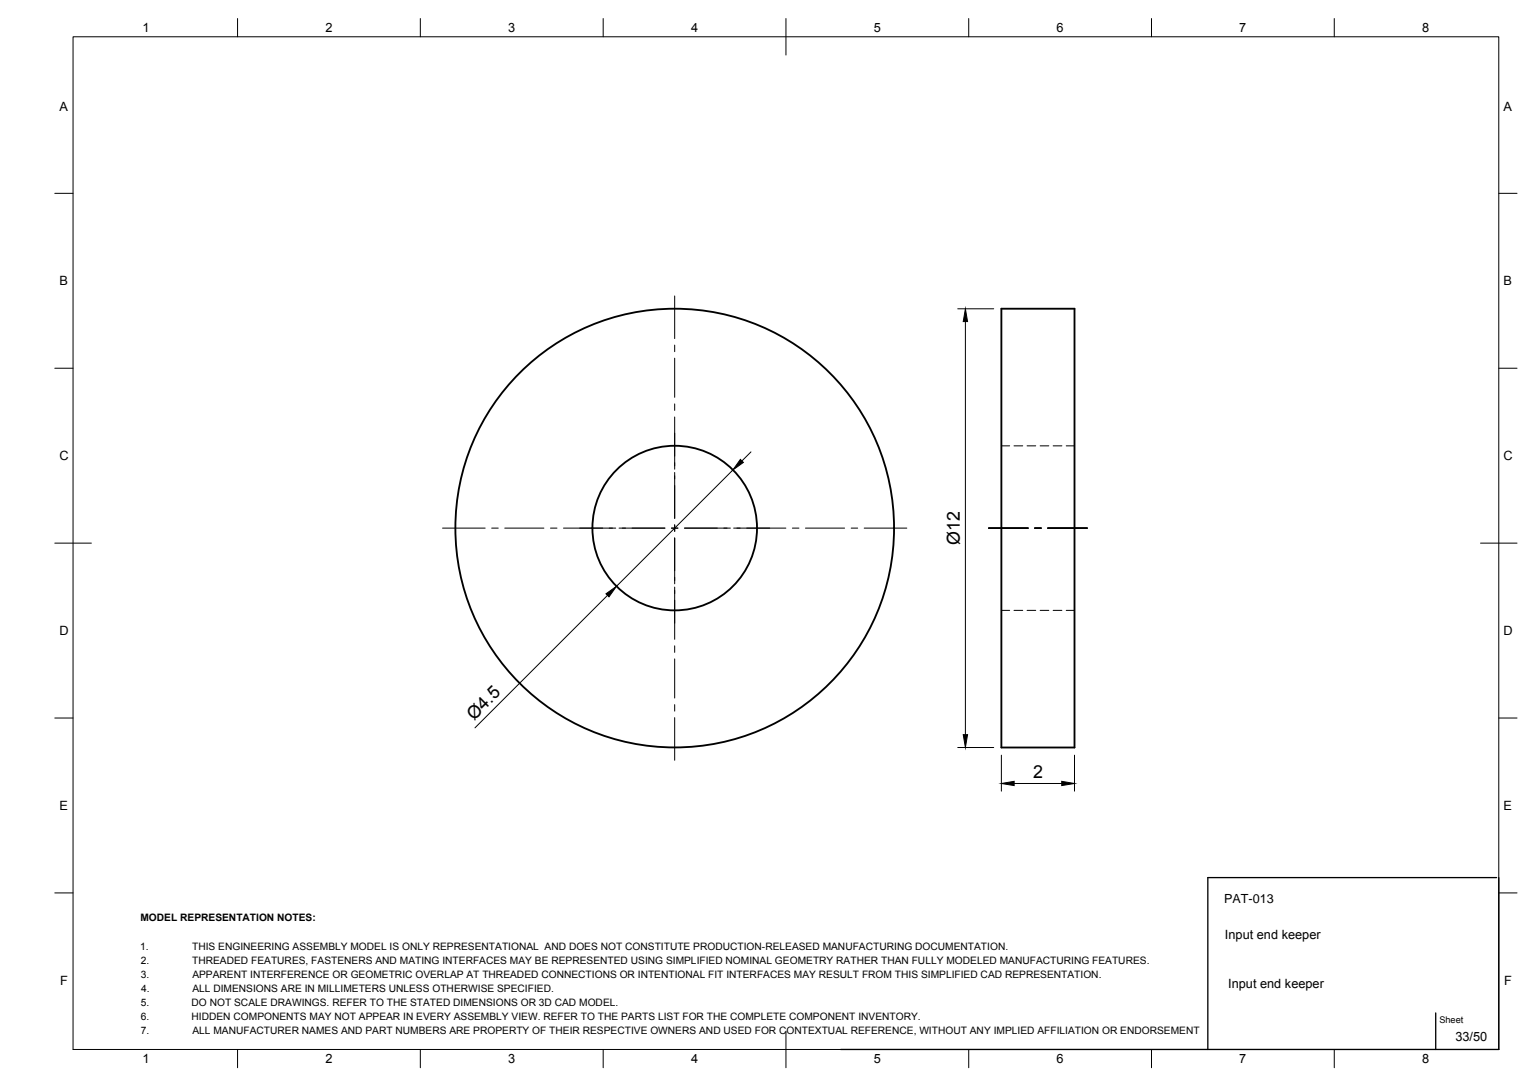
ISO-10303-21;
HEADER;
/* Generated by software containing ST-Developer
 * from STEP Tools, Inc. (www.steptools.com) 
 */

FILE_DESCRIPTION(
/* description */ ('Belt-driven linear axis on 2020 extrusion'),
/* implementation_level */ '2;1');

FILE_NAME(
/* name */ 'Input end keeper.step',
/* time_stamp */ '2026-10-28T03:26:09-07:00',
/* author */ (''),
/* organization */ (''),
/* preprocessor_version */ 'ST-DEVELOPER v20.2',
/* originating_system */ 'Autodesk Translation Framework v15.17.0.0',
/* authorisation */ '');

FILE_SCHEMA (('AUTOMOTIVE_DESIGN { 1 0 10303 214 3 1 1 }'));
ENDSEC;

DATA;
#10=MECHANICAL_DESIGN_GEOMETRIC_PRESENTATION_REPRESENTATION('',(#648),#20096);
#546=SHAPE_REPRESENTATION_RELATIONSHIP('SRR','None',#20344,#592);
#592=ADVANCED_BREP_SHAPE_REPRESENTATION('',(#703),#20075);
#648=STYLED_ITEM('',(#20643),#703);
#703=MANIFOLD_SOLID_BREP('Body1',#10962);
#838=FACE_BOUND('',#2390,.T.);
#839=FACE_BOUND('',#2392,.T.);
#1125=PLANE('',#12252);
#1126=PLANE('',#12253);
#1645=FACE_OUTER_BOUND('',#2387,.T.);
#1646=FACE_OUTER_BOUND('',#2388,.T.);
#1647=FACE_OUTER_BOUND('',#2389,.T.);
#1648=FACE_OUTER_BOUND('',#2391,.T.);
#2387=EDGE_LOOP('',(#9037,#9038,#9039,#9040));
#2388=EDGE_LOOP('',(#9041,#9042,#9043,#9044));
#2389=EDGE_LOOP('',(#9045));
#2390=EDGE_LOOP('',(#9046));
#2391=EDGE_LOOP('',(#9047));
#2392=EDGE_LOOP('',(#9048));
#3216=LINE('',#18502,#4073);
#3217=LINE('',#18508,#4074);
#4073=VECTOR('',#14852,0.225);
#4074=VECTOR('',#14859,0.6);
#4700=CIRCLE('',#12247,0.225);
#4701=CIRCLE('',#12248,0.225);
#4702=CIRCLE('',#12250,0.6);
#4703=CIRCLE('',#12251,0.6);
#5495=VERTEX_POINT('',#18499);
#5496=VERTEX_POINT('',#18501);
#5497=VERTEX_POINT('',#18505);
#5498=VERTEX_POINT('',#18507);
#6733=EDGE_CURVE('',#5495,#5495,#4700,.T.);
#6734=EDGE_CURVE('',#5495,#5496,#3216,.T.);
#6735=EDGE_CURVE('',#5496,#5496,#4701,.T.);
#6736=EDGE_CURVE('',#5497,#5497,#4702,.T.);
#6737=EDGE_CURVE('',#5497,#5498,#3217,.T.);
#6738=EDGE_CURVE('',#5498,#5498,#4703,.T.);
#9037=ORIENTED_EDGE('',*,*,#6733,.F.);
#9038=ORIENTED_EDGE('',*,*,#6734,.T.);
#9039=ORIENTED_EDGE('',*,*,#6735,.T.);
#9040=ORIENTED_EDGE('',*,*,#6734,.F.);
#9041=ORIENTED_EDGE('',*,*,#6736,.F.);
#9042=ORIENTED_EDGE('',*,*,#6737,.T.);
#9043=ORIENTED_EDGE('',*,*,#6738,.T.);
#9044=ORIENTED_EDGE('',*,*,#6737,.F.);
#9045=ORIENTED_EDGE('',*,*,#6736,.T.);
#9046=ORIENTED_EDGE('',*,*,#6733,.T.);
#9047=ORIENTED_EDGE('',*,*,#6738,.F.);
#9048=ORIENTED_EDGE('',*,*,#6735,.F.);
#10211=CYLINDRICAL_SURFACE('',#12246,0.225);
#10212=CYLINDRICAL_SURFACE('',#12249,0.6);
#10696=ADVANCED_FACE('',(#1645),#10211,.F.);
#10697=ADVANCED_FACE('',(#1646),#10212,.T.);
#10698=ADVANCED_FACE('',(#1647,#838),#1125,.T.);
#10699=ADVANCED_FACE('',(#1648,#839),#1126,.F.);
#10962=CLOSED_SHELL('',(#10696,#10697,#10698,#10699));
#12245=AXIS2_PLACEMENT_3D('',#18497,#14846,#14847);
#12246=AXIS2_PLACEMENT_3D('',#18498,#14848,#14849);
#12247=AXIS2_PLACEMENT_3D('',#18500,#14850,#14851);
#12248=AXIS2_PLACEMENT_3D('',#18503,#14853,#14854);
#12249=AXIS2_PLACEMENT_3D('',#18504,#14855,#14856);
#12250=AXIS2_PLACEMENT_3D('',#18506,#14857,#14858);
#12251=AXIS2_PLACEMENT_3D('',#18509,#14860,#14861);
#12252=AXIS2_PLACEMENT_3D('',#18510,#14862,#14863);
#12253=AXIS2_PLACEMENT_3D('',#18511,#14864,#14865);
#14846=DIRECTION('axis',(0.,0.,1.));
#14847=DIRECTION('refdir',(1.,0.,0.));
#14848=DIRECTION('center_axis',(0.,1.,0.));
#14849=DIRECTION('ref_axis',(1.,0.,0.));
#14850=DIRECTION('center_axis',(0.,-1.,0.));
#14851=DIRECTION('ref_axis',(1.,0.,0.));
#14852=DIRECTION('',(0.,-1.,0.));
#14853=DIRECTION('center_axis',(0.,-1.,0.));
#14854=DIRECTION('ref_axis',(1.,0.,0.));
#14855=DIRECTION('center_axis',(0.,1.,0.));
#14856=DIRECTION('ref_axis',(1.,0.,0.));
#14857=DIRECTION('center_axis',(0.,1.,0.));
#14858=DIRECTION('ref_axis',(1.,0.,0.));
#14859=DIRECTION('',(0.,-1.,0.));
#14860=DIRECTION('center_axis',(0.,1.,0.));
#14861=DIRECTION('ref_axis',(1.,0.,0.));
#14862=DIRECTION('center_axis',(0.,1.,0.));
#14863=DIRECTION('ref_axis',(1.,0.,0.));
#14864=DIRECTION('center_axis',(0.,1.,0.));
#14865=DIRECTION('ref_axis',(1.,0.,0.));
#18497=CARTESIAN_POINT('',(0.,0.,0.));
#18498=CARTESIAN_POINT('Origin',(0.,-5.2,7.));
#18499=CARTESIAN_POINT('',(-0.225,-5.,7.));
#18500=CARTESIAN_POINT('Origin',(0.,-5.,7.));
#18501=CARTESIAN_POINT('',(-0.225,-5.2,7.));
#18502=CARTESIAN_POINT('',(-0.225,-5.2,7.));
#18503=CARTESIAN_POINT('Origin',(0.,-5.2,7.));
#18504=CARTESIAN_POINT('Origin',(0.,-5.2,7.));
#18505=CARTESIAN_POINT('',(-0.6,-5.,7.));
#18506=CARTESIAN_POINT('Origin',(0.,-5.,7.));
#18507=CARTESIAN_POINT('',(-0.6,-5.2,7.));
#18508=CARTESIAN_POINT('',(-0.6,-5.2,7.));
#18509=CARTESIAN_POINT('Origin',(0.,-5.2,7.));
#18510=CARTESIAN_POINT('Origin',(0.,-5.,7.));
#18511=CARTESIAN_POINT('Origin',(0.,-5.2,7.));
#20021=UNCERTAINTY_MEASURE_WITH_UNIT(LENGTH_MEASURE(0.001),#20097,
'DISTANCE_ACCURACY_VALUE',
'Maximum model space distance between geometric entities at asserted c
onnectivities');
#20042=UNCERTAINTY_MEASURE_WITH_UNIT(LENGTH_MEASURE(0.001),#20097,
'DISTANCE_ACCURACY_VALUE',
'Maximum model space distance between geometric entities at asserted c
onnectivities');
#20075=(
GEOMETRIC_REPRESENTATION_CONTEXT(3)
GLOBAL_UNCERTAINTY_ASSIGNED_CONTEXT((#20021))
GLOBAL_UNIT_ASSIGNED_CONTEXT((#20097,#20099,#20100))
REPRESENTATION_CONTEXT('','3D')
);
#20096=(
GEOMETRIC_REPRESENTATION_CONTEXT(3)
GLOBAL_UNCERTAINTY_ASSIGNED_CONTEXT((#20042))
GLOBAL_UNIT_ASSIGNED_CONTEXT((#20097,#20099,#20100))
REPRESENTATION_CONTEXT('','3D')
);
#20097=(
LENGTH_UNIT()
NAMED_UNIT(*)
SI_UNIT(.CENTI.,.METRE.)
);
#20099=(
NAMED_UNIT(*)
PLANE_ANGLE_UNIT()
SI_UNIT($,.RADIAN.)
);
#20100=(
NAMED_UNIT(*)
SI_UNIT($,.STERADIAN.)
SOLID_ANGLE_UNIT()
);
#20133=SHAPE_DEFINITION_REPRESENTATION(#20191,#20344);
#20191=PRODUCT_DEFINITION_SHAPE('',$,#20398);
#20344=SHAPE_REPRESENTATION('',(#12245),#20075);
#20365=PRODUCT_DEFINITION_CONTEXT('part definition',#20526,'design');
#20398=PRODUCT_DEFINITION('Input end keeper','Input end keeper',#20451,
#20365);
#20451=PRODUCT_DEFINITION_FORMATION('',$,#20560);
#20526=APPLICATION_CONTEXT(
'Core Data for Automotive Mechanical Design Process');
#20527=PRODUCT_CONTEXT('part definition',#20526,'mechanical');
#20560=PRODUCT('Input end keeper','Input end keeper','Input end keeper',
(#20527));
#20637=COLOUR_RGB('Sky Blue',0.24,0.69,0.87);
#20638=FILL_AREA_STYLE_COLOUR('',#20637);
#20639=FILL_AREA_STYLE('',(#20638));
#20640=SURFACE_STYLE_FILL_AREA(#20639);
#20641=SURFACE_SIDE_STYLE('',(#20640));
#20642=SURFACE_STYLE_USAGE(.BOTH.,#20641);
#20643=PRESENTATION_STYLE_ASSIGNMENT((#20642));
ENDSEC;
END-ISO-10303-21;
